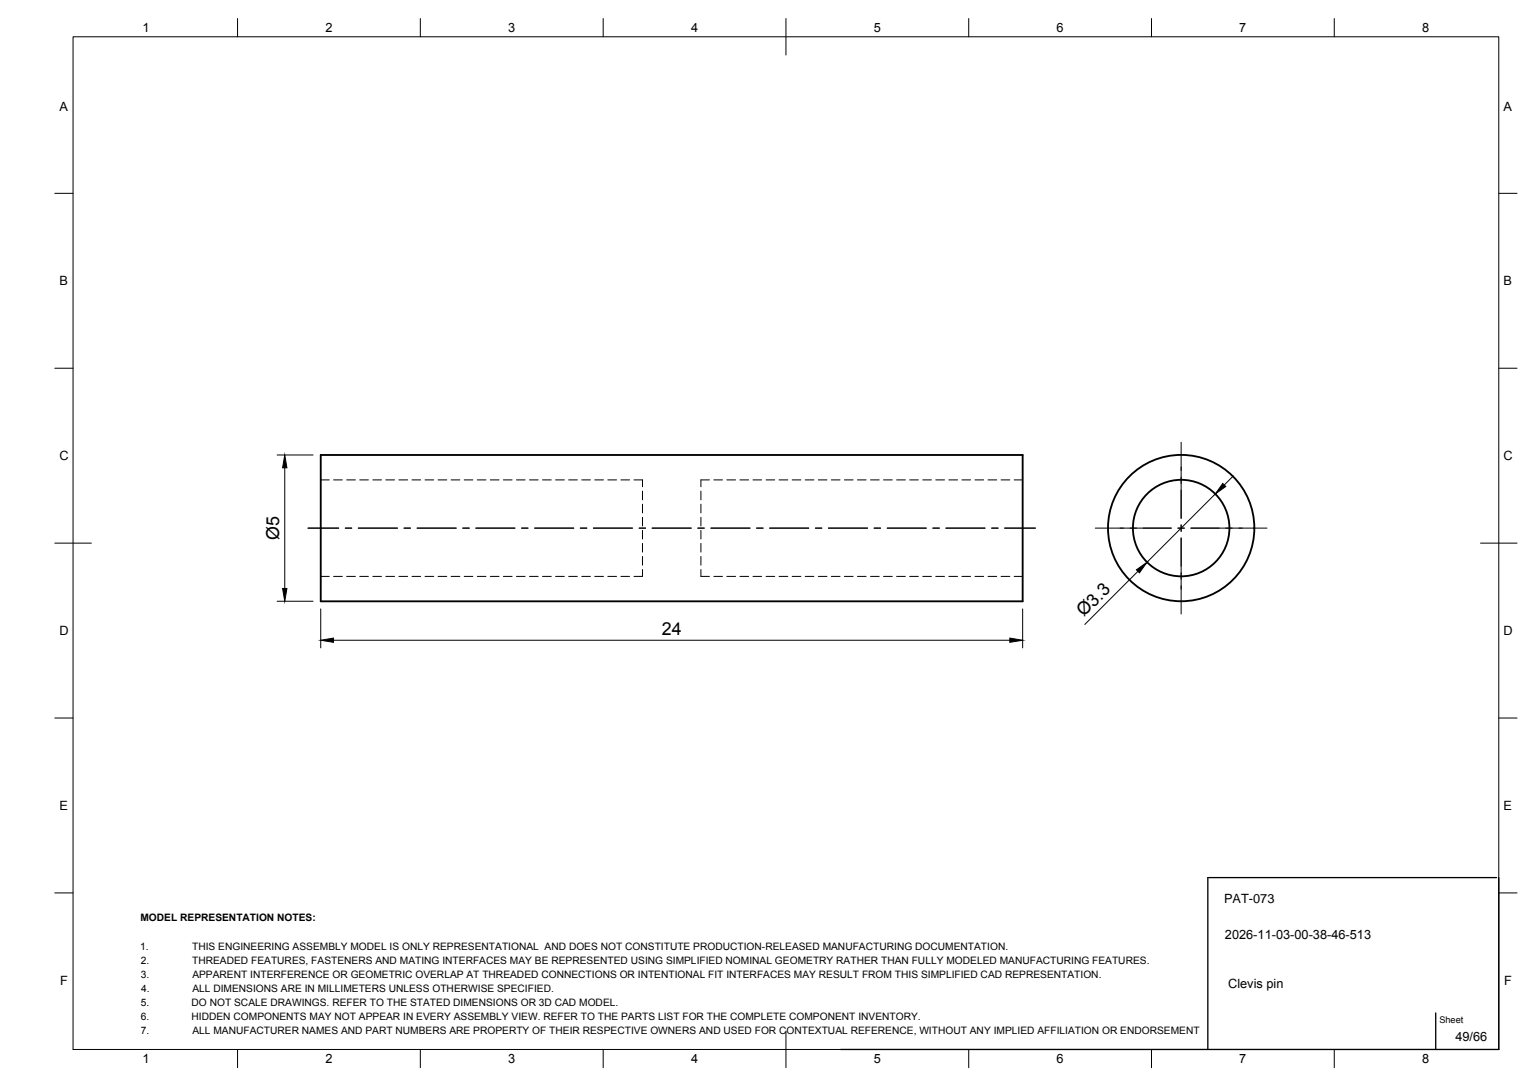
ISO-10303-21;
HEADER;
/* Generated by software containing ST-Developer
 * from STEP Tools, Inc. (www.steptools.com) 
 */

FILE_DESCRIPTION(
/* description */ ('Manual piston pump'),
/* implementation_level */ '2;1');

FILE_NAME(
/* name */ 'Clevis pin.step',
/* time_stamp */ '2026-11-02T16:54:23-08:00',
/* author */ (''),
/* organization */ (''),
/* preprocessor_version */ 'ST-DEVELOPER v20.2',
/* originating_system */ 'Autodesk Translation Framework v15.17.0.0',
/* authorisation */ '');

FILE_SCHEMA (('AUTOMOTIVE_DESIGN { 1 0 10303 214 3 1 1 }'));
ENDSEC;

DATA;
#10=MECHANICAL_DESIGN_GEOMETRIC_PRESENTATION_REPRESENTATION('',(#740),#19043);
#606=SHAPE_REPRESENTATION_RELATIONSHIP('SRR','None',#19355,#669);
#669=ADVANCED_BREP_SHAPE_REPRESENTATION('',(#809),#19022);
#740=STYLED_ITEM('',(#19661),#809);
#809=MANIFOLD_SOLID_BREP('Body1',#9527);
#1013=FACE_BOUND('',#2498,.T.);
#1014=FACE_BOUND('',#2500,.T.);
#1247=CYLINDRICAL_SURFACE('',#11129,0.165);
#1248=CYLINDRICAL_SURFACE('',#11133,0.165);
#1249=CYLINDRICAL_SURFACE('',#11137,0.25);
#1731=FACE_OUTER_BOUND('',#2492,.T.);
#1732=FACE_OUTER_BOUND('',#2493,.T.);
#1733=FACE_OUTER_BOUND('',#2494,.T.);
#1734=FACE_OUTER_BOUND('',#2495,.T.);
#1735=FACE_OUTER_BOUND('',#2496,.T.);
#1736=FACE_OUTER_BOUND('',#2497,.T.);
#1737=FACE_OUTER_BOUND('',#2499,.T.);
#2492=EDGE_LOOP('',(#8061,#8062,#8063,#8064));
#2493=EDGE_LOOP('',(#8065));
#2494=EDGE_LOOP('',(#8066,#8067,#8068,#8069));
#2495=EDGE_LOOP('',(#8070));
#2496=EDGE_LOOP('',(#8071,#8072,#8073,#8074));
#2497=EDGE_LOOP('',(#8075));
#2498=EDGE_LOOP('',(#8076));
#2499=EDGE_LOOP('',(#8077));
#2500=EDGE_LOOP('',(#8078));
#3048=CIRCLE('',#11130,0.165);
#3049=CIRCLE('',#11131,0.165);
#3050=CIRCLE('',#11134,0.165);
#3051=CIRCLE('',#11135,0.165);
#3052=CIRCLE('',#11138,0.25);
#3053=CIRCLE('',#11139,0.25);
#3608=LINE('',#18106,#4212);
#3609=LINE('',#18113,#4213);
#3610=LINE('',#18120,#4214);
#4212=VECTOR('',#13732,0.165);
#4213=VECTOR('',#13741,0.165);
#4214=VECTOR('',#13750,0.25);
#4956=VERTEX_POINT('',#18103);
#4957=VERTEX_POINT('',#18105);
#4958=VERTEX_POINT('',#18110);
#4959=VERTEX_POINT('',#18112);
#4960=VERTEX_POINT('',#18117);
#4961=VERTEX_POINT('',#18119);
#6017=EDGE_CURVE('',#4956,#4956,#3048,.T.);
#6018=EDGE_CURVE('',#4956,#4957,#3608,.T.);
#6019=EDGE_CURVE('',#4957,#4957,#3049,.T.);
#6020=EDGE_CURVE('',#4958,#4958,#3050,.T.);
#6021=EDGE_CURVE('',#4958,#4959,#3609,.T.);
#6022=EDGE_CURVE('',#4959,#4959,#3051,.T.);
#6023=EDGE_CURVE('',#4960,#4960,#3052,.T.);
#6024=EDGE_CURVE('',#4960,#4961,#3610,.T.);
#6025=EDGE_CURVE('',#4961,#4961,#3053,.T.);
#8061=ORIENTED_EDGE('',*,*,#6017,.F.);
#8062=ORIENTED_EDGE('',*,*,#6018,.T.);
#8063=ORIENTED_EDGE('',*,*,#6019,.F.);
#8064=ORIENTED_EDGE('',*,*,#6018,.F.);
#8065=ORIENTED_EDGE('',*,*,#6017,.T.);
#8066=ORIENTED_EDGE('',*,*,#6020,.F.);
#8067=ORIENTED_EDGE('',*,*,#6021,.T.);
#8068=ORIENTED_EDGE('',*,*,#6022,.T.);
#8069=ORIENTED_EDGE('',*,*,#6021,.F.);
#8070=ORIENTED_EDGE('',*,*,#6022,.F.);
#8071=ORIENTED_EDGE('',*,*,#6023,.F.);
#8072=ORIENTED_EDGE('',*,*,#6024,.T.);
#8073=ORIENTED_EDGE('',*,*,#6025,.T.);
#8074=ORIENTED_EDGE('',*,*,#6024,.F.);
#8075=ORIENTED_EDGE('',*,*,#6023,.T.);
#8076=ORIENTED_EDGE('',*,*,#6019,.T.);
#8077=ORIENTED_EDGE('',*,*,#6025,.F.);
#8078=ORIENTED_EDGE('',*,*,#6020,.T.);
#8815=PLANE('',#11132);
#8816=PLANE('',#11136);
#8817=PLANE('',#11140);
#8818=PLANE('',#11141);
#9336=ADVANCED_FACE('',(#1731),#1247,.F.);
#9337=ADVANCED_FACE('',(#1732),#8815,.T.);
#9338=ADVANCED_FACE('',(#1733),#1248,.F.);
#9339=ADVANCED_FACE('',(#1734),#8816,.F.);
#9340=ADVANCED_FACE('',(#1735),#1249,.T.);
#9341=ADVANCED_FACE('',(#1736,#1013),#8817,.T.);
#9342=ADVANCED_FACE('',(#1737,#1014),#8818,.F.);
#9527=CLOSED_SHELL('',(#9336,#9337,#9338,#9339,#9340,#9341,#9342));
#11128=AXIS2_PLACEMENT_3D('',#18101,#13726,#13727);
#11129=AXIS2_PLACEMENT_3D('',#18102,#13728,#13729);
#11130=AXIS2_PLACEMENT_3D('',#18104,#13730,#13731);
#11131=AXIS2_PLACEMENT_3D('',#18107,#13733,#13734);
#11132=AXIS2_PLACEMENT_3D('',#18108,#13735,#13736);
#11133=AXIS2_PLACEMENT_3D('',#18109,#13737,#13738);
#11134=AXIS2_PLACEMENT_3D('',#18111,#13739,#13740);
#11135=AXIS2_PLACEMENT_3D('',#18114,#13742,#13743);
#11136=AXIS2_PLACEMENT_3D('',#18115,#13744,#13745);
#11137=AXIS2_PLACEMENT_3D('',#18116,#13746,#13747);
#11138=AXIS2_PLACEMENT_3D('',#18118,#13748,#13749);
#11139=AXIS2_PLACEMENT_3D('',#18121,#13751,#13752);
#11140=AXIS2_PLACEMENT_3D('',#18122,#13753,#13754);
#11141=AXIS2_PLACEMENT_3D('',#18123,#13755,#13756);
#13726=DIRECTION('axis',(0.,0.,1.));
#13727=DIRECTION('refdir',(1.,0.,0.));
#13728=DIRECTION('center_axis',(1.,0.,0.));
#13729=DIRECTION('ref_axis',(0.,0.,-1.));
#13730=DIRECTION('center_axis',(1.,0.,0.));
#13731=DIRECTION('ref_axis',(0.,0.,-1.));
#13732=DIRECTION('',(1.,0.,0.));
#13733=DIRECTION('center_axis',(-1.,0.,0.));
#13734=DIRECTION('ref_axis',(0.,0.,-1.));
#13735=DIRECTION('center_axis',(1.,0.,0.));
#13736=DIRECTION('ref_axis',(0.,0.,-1.));
#13737=DIRECTION('center_axis',(1.,0.,0.));
#13738=DIRECTION('ref_axis',(0.,0.,-1.));
#13739=DIRECTION('center_axis',(1.,0.,0.));
#13740=DIRECTION('ref_axis',(0.,0.,-1.));
#13741=DIRECTION('',(1.,0.,0.));
#13742=DIRECTION('center_axis',(1.,0.,0.));
#13743=DIRECTION('ref_axis',(0.,0.,-1.));
#13744=DIRECTION('center_axis',(1.,0.,0.));
#13745=DIRECTION('ref_axis',(0.,0.,-1.));
#13746=DIRECTION('center_axis',(1.,0.,0.));
#13747=DIRECTION('ref_axis',(0.,0.,-1.));
#13748=DIRECTION('center_axis',(1.,0.,0.));
#13749=DIRECTION('ref_axis',(0.,0.,-1.));
#13750=DIRECTION('',(-1.,0.,0.));
#13751=DIRECTION('center_axis',(1.,0.,0.));
#13752=DIRECTION('ref_axis',(0.,0.,-1.));
#13753=DIRECTION('center_axis',(1.,0.,0.));
#13754=DIRECTION('ref_axis',(0.,0.,-1.));
#13755=DIRECTION('center_axis',(1.,0.,0.));
#13756=DIRECTION('ref_axis',(0.,0.,-1.));
#18101=CARTESIAN_POINT('',(0.,0.,0.));
#18102=CARTESIAN_POINT('Origin',(0.1,-6.1,4.5));
#18103=CARTESIAN_POINT('',(0.1,-6.1,4.665));
#18104=CARTESIAN_POINT('Origin',(0.1,-6.1,4.5));
#18105=CARTESIAN_POINT('',(1.2,-6.1,4.665));
#18106=CARTESIAN_POINT('',(0.1,-6.1,4.665));
#18107=CARTESIAN_POINT('Origin',(1.2,-6.1,4.5));
#18108=CARTESIAN_POINT('Origin',(0.1,-6.1,4.5));
#18109=CARTESIAN_POINT('Origin',(-1.3,-6.1,4.5));
#18110=CARTESIAN_POINT('',(-1.2,-6.1,4.665));
#18111=CARTESIAN_POINT('Origin',(-1.2,-6.1,4.5));
#18112=CARTESIAN_POINT('',(-0.0999999999999999,-6.1,4.665));
#18113=CARTESIAN_POINT('',(-1.3,-6.1,4.665));
#18114=CARTESIAN_POINT('Origin',(-0.0999999999999999,-6.1,4.5));
#18115=CARTESIAN_POINT('Origin',(-0.0999999999999999,-6.1,4.5));
#18116=CARTESIAN_POINT('Origin',(-1.2,-6.1,4.5));
#18117=CARTESIAN_POINT('',(1.2,-6.1,4.75));
#18118=CARTESIAN_POINT('Origin',(1.2,-6.1,4.5));
#18119=CARTESIAN_POINT('',(-1.2,-6.1,4.75));
#18120=CARTESIAN_POINT('',(-1.2,-6.1,4.75));
#18121=CARTESIAN_POINT('Origin',(-1.2,-6.1,4.5));
#18122=CARTESIAN_POINT('Origin',(1.2,-6.1,4.5));
#18123=CARTESIAN_POINT('Origin',(-1.2,-6.1,4.5));
#18951=UNCERTAINTY_MEASURE_WITH_UNIT(LENGTH_MEASURE(0.001),#19044,
'DISTANCE_ACCURACY_VALUE',
'Maximum model space distance between geometric entities at asserted c
onnectivities');
#18972=UNCERTAINTY_MEASURE_WITH_UNIT(LENGTH_MEASURE(0.001),#19044,
'DISTANCE_ACCURACY_VALUE',
'Maximum model space distance between geometric entities at asserted c
onnectivities');
#19022=(
GEOMETRIC_REPRESENTATION_CONTEXT(3)
GLOBAL_UNCERTAINTY_ASSIGNED_CONTEXT((#18951))
GLOBAL_UNIT_ASSIGNED_CONTEXT((#19044,#19046,#19047))
REPRESENTATION_CONTEXT('','3D')
);
#19043=(
GEOMETRIC_REPRESENTATION_CONTEXT(3)
GLOBAL_UNCERTAINTY_ASSIGNED_CONTEXT((#18972))
GLOBAL_UNIT_ASSIGNED_CONTEXT((#19044,#19046,#19047))
REPRESENTATION_CONTEXT('','3D')
);
#19044=(
LENGTH_UNIT()
NAMED_UNIT(*)
SI_UNIT(.CENTI.,.METRE.)
);
#19046=(
NAMED_UNIT(*)
PLANE_ANGLE_UNIT()
SI_UNIT($,.RADIAN.)
);
#19047=(
NAMED_UNIT(*)
SI_UNIT($,.STERADIAN.)
SOLID_ANGLE_UNIT()
);
#19097=SHAPE_DEFINITION_REPRESENTATION(#19174,#19355);
#19174=PRODUCT_DEFINITION_SHAPE('',$,#19426);
#19355=SHAPE_REPRESENTATION('',(#11128),#19022);
#19376=PRODUCT_DEFINITION_CONTEXT('part definition',#19588,'design');
#19426=PRODUCT_DEFINITION('2026-11-03-00-38-46-513','Clevis pin',#19496,
#19376);
#19496=PRODUCT_DEFINITION_FORMATION('',$,#19639);
#19588=APPLICATION_CONTEXT(
'Core Data for Automotive Mechanical Design Process');
#19589=PRODUCT_CONTEXT('part definition',#19588,'mechanical');
#19639=PRODUCT('2026-11-03-00-38-46-513','Clevis pin','Clevis pin',(#19589));
#19661=PRESENTATION_STYLE_ASSIGNMENT((#19667));
#19667=SURFACE_STYLE_USAGE(.BOTH.,#19673);
#19673=SURFACE_SIDE_STYLE('',(#19679));
#19679=SURFACE_STYLE_FILL_AREA(#19685);
#19685=FILL_AREA_STYLE('CAD Library Painted - Engineering blue',(#19691));
#19691=FILL_AREA_STYLE_COLOUR('CAD Library Painted - Engineering blue',
#19697);
#19697=COLOUR_RGB('CAD Library Painted - Engineering blue',0.12156862745098,
0.356862745098039,0.6);
ENDSEC;
END-ISO-10303-21;
